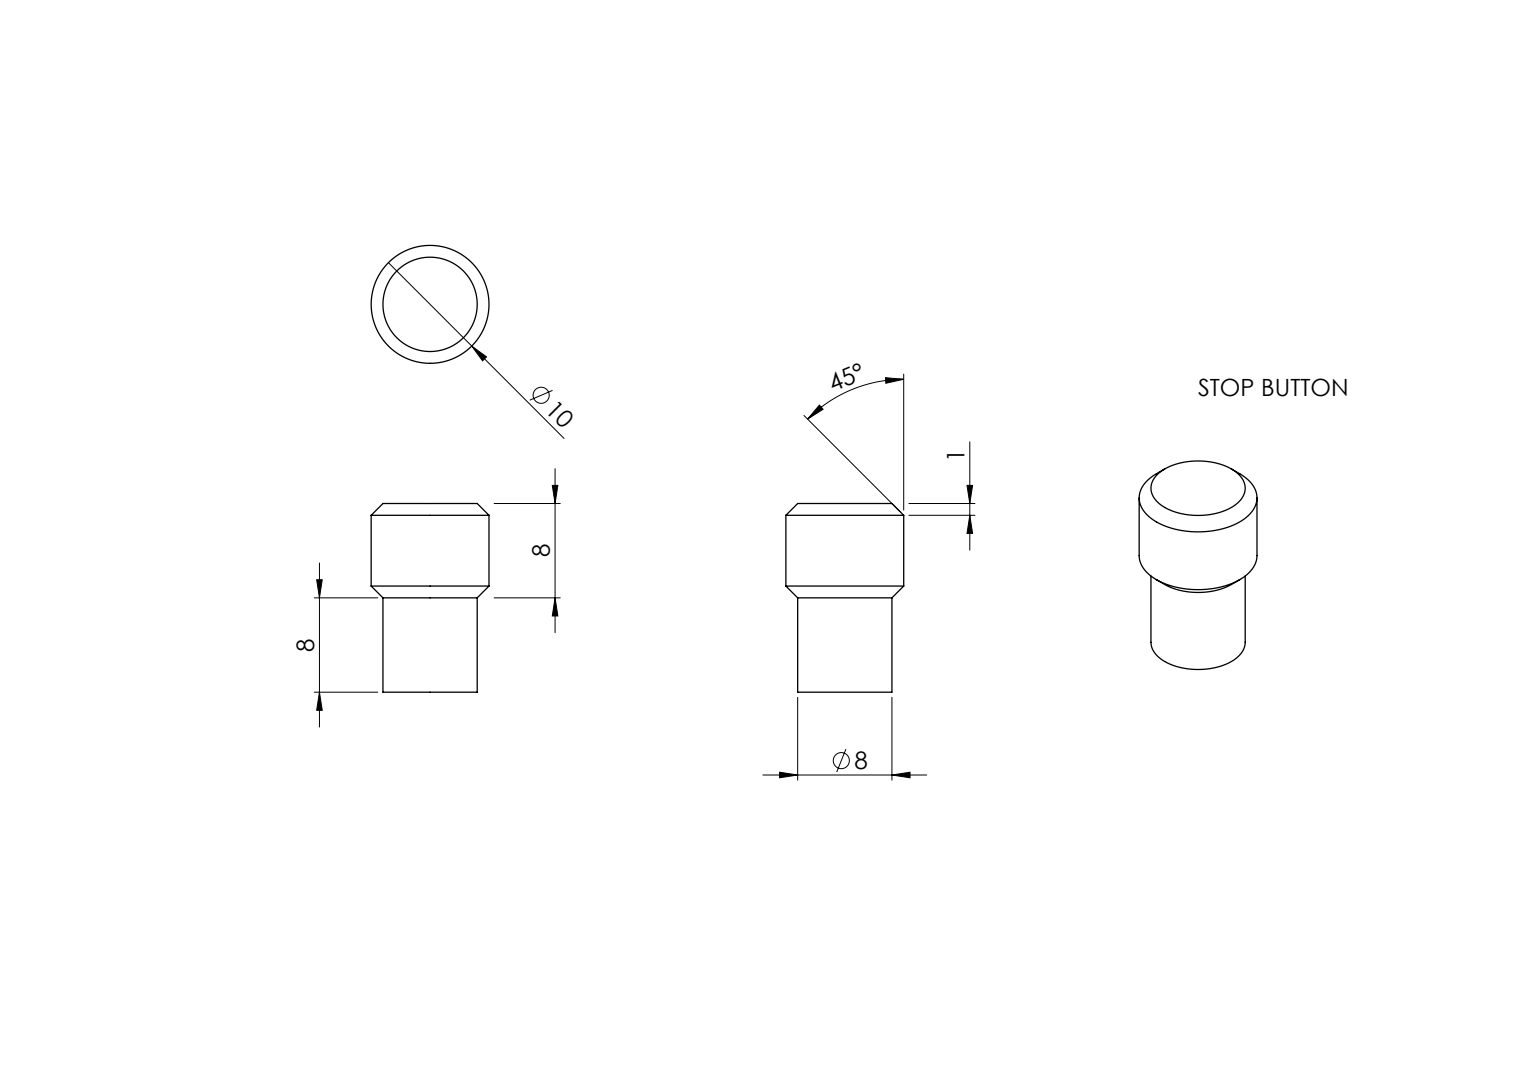
ISO-10303-21;
HEADER;
FILE_DESCRIPTION (('STEP AP214'),
    '1' );
FILE_NAME ('stop button.step',
    '2026-10-26T11:20:31',
    ( '' ),
    ( '' ),
    'SwSTEP 2.0',
    'SolidWorks 2026',
    '' );
FILE_SCHEMA (( 'AUTOMOTIVE_DESIGN' ));
ENDSEC;

DATA;
#2=ORIENTED_EDGE ( 'NONE', *, *, #1110, .F. ) ;
#22=VERTEX_POINT ( 'NONE', #4223 ) ;
#32=( LENGTH_UNIT ( ) NAMED_UNIT ( * ) SI_UNIT ( .MILLI., .METRE. ) );
#39=CIRCLE ( 'NONE', #1106, 4.000000000000000000 ) ;
#62=DIRECTION ( 'NONE',  ( 0.000000000000000000, 0.000000000000000000, 1.000000000000000000 ) ) ;
#65=DIRECTION ( 'NONE',  ( 0.000000000000000000, 1.000000000000000000, 0.000000000000000000 ) ) ;
#85=VERTEX_POINT ( 'NONE', #4577 ) ;
#123=DIRECTION ( 'NONE',  ( -0.000000000000000000, -1.000000000000000000, -0.000000000000000000 ) ) ;
#130=DIRECTION ( 'NONE',  ( 0.000000000000000000, 0.000000000000000000, 1.000000000000000000 ) ) ;
#135=PRODUCT_DEFINITION_FORMATION_WITH_SPECIFIED_SOURCE ( 'ANY', '', #1681, .NOT_KNOWN. ) ;
#149=ORIENTED_EDGE ( 'NONE', *, *, #4614, .F. ) ;
#153=UNCERTAINTY_MEASURE_WITH_UNIT (LENGTH_MEASURE( 1.000000000000000082E-05 ), #374, 'distance_accuracy_value', 'NONE');
#173=CIRCLE ( 'NONE', #776, 5.000000000000000888 ) ;
#201=FACE_OUTER_BOUND ( 'NONE', #427, .T. ) ;
#205=AXIS2_PLACEMENT_3D ( 'NONE', #2218, #4537, #1354 ) ;
#255=DIRECTION ( 'NONE',  ( 0.000000000000000000, 0.000000000000000000, 1.000000000000000000 ) ) ;
#282=ORIENTED_EDGE ( 'NONE', *, *, #4614, .T. ) ;
#288=PRODUCT_DEFINITION_CONTEXT ( 'detailed design', #920, 'design' ) ;
#308=CARTESIAN_POINT ( 'NONE',  ( 3.469446951953614189E-15, 34.00000000000000000, 8.999999999999992895 ) ) ;
#310=VERTEX_POINT ( 'NONE', #3063 ) ;
#320=PRODUCT_CONTEXT ( 'NONE', #3923, 'mechanical' ) ;
#323=DIRECTION ( 'NONE',  ( -0.000000000000000000, -1.000000000000000000, -0.000000000000000000 ) ) ;
#324=LINE ( 'NONE', #1796, #4294 ) ;
#352=CARTESIAN_POINT ( 'NONE',  ( 3.469446951953614189E-15, 41.00000000000000000, 8.999999999999992895 ) ) ;
#374=( LENGTH_UNIT ( ) NAMED_UNIT ( * ) SI_UNIT ( .MILLI., .METRE. ) );
#380=AXIS2_PLACEMENT_3D ( 'NONE', #2484, #3587, #1024 ) ;
#385=CARTESIAN_POINT ( 'NONE',  ( 3.469446951953614189E-15, 33.00000000000000000, 8.999999999999992895 ) ) ;
#397=( NAMED_UNIT ( * ) SI_UNIT ( $, .STERADIAN. ) SOLID_ANGLE_UNIT ( ) );
#403=DIRECTION ( 'NONE',  ( -0.000000000000000000, 1.000000000000000000, -0.000000000000000000 ) ) ;
#427=EDGE_LOOP ( 'NONE', ( #1515, #2000, #282, #1851 ) ) ;
#450=ORIENTED_EDGE ( 'NONE', *, *, #688, .F. ) ;
#473=SURFACE_STYLE_FILL_AREA ( #1539 ) ;
#578=( GEOMETRIC_REPRESENTATION_CONTEXT ( 3 ) GLOBAL_UNCERTAINTY_ASSIGNED_CONTEXT ( ( #4075 ) ) GLOBAL_UNIT_ASSIGNED_CONTEXT ( ( #32, #1473, #1933 ) ) REPRESENTATION_CONTEXT ( 'NONE', 'WORKASPACE' ) );
#580=DIRECTION ( 'NONE',  ( 0.000000000000000000, 1.000000000000000000, 0.000000000000000000 ) ) ;
#584=DIRECTION ( 'NONE',  ( -0.000000000000000000, -1.000000000000000000, -0.000000000000000000 ) ) ;
#592=MECHANICAL_DESIGN_GEOMETRIC_PRESENTATION_REPRESENTATION('',(#1718),#2469);
#617=DIRECTION ( 'NONE',  ( 0.000000000000000000, 0.000000000000000000, 1.000000000000000000 ) ) ;
#642=CARTESIAN_POINT ( 'NONE',  ( 3.469446951953614189E-15, 37.00000000000000711, 4.999999999999992006 ) ) ;
#688=EDGE_CURVE ( 'NONE', #2966, #22, #4307, .T. ) ;
#697=LINE ( 'NONE', #3186, #1821 ) ;
#759=ORIENTED_EDGE ( 'NONE', *, *, #4685, .T. ) ;
#776=AXIS2_PLACEMENT_3D ( 'NONE', #3918, #3873, #255 ) ;
#804=EDGE_CURVE ( 'NONE', #85, #3729, #1345, .T. ) ;
#865=DIRECTION ( 'NONE',  ( -0.000000000000000000, 1.000000000000000000, -0.000000000000000000 ) ) ;
#912=CARTESIAN_POINT ( 'NONE',  ( 3.469446951953614189E-15, 25.00000000000000000, 8.999999999999992895 ) ) ;
#916=EDGE_CURVE ( 'NONE', #22, #310, #1522, .T. ) ;
#920=APPLICATION_CONTEXT ( 'automotive_design' ) ;
#946=CYLINDRICAL_SURFACE ( 'NONE', #2530, 5.000000000000000888 ) ;
#957=ADVANCED_FACE ( 'NONE', ( #3302 ), #1952, .T. ) ;
#1002=DIRECTION ( 'NONE',  ( -0.000000000000000000, -1.000000000000000000, -0.000000000000000000 ) ) ;
#1021=ORIENTED_EDGE ( 'NONE', *, *, #4190, .F. ) ;
#1024=DIRECTION ( 'NONE',  ( 0.000000000000000000, -0.000000000000000000, 1.000000000000000000 ) ) ;
#1040=EDGE_CURVE ( 'NONE', #2780, #85, #1094, .T. ) ;
#1084=AXIS2_PLACEMENT_3D ( 'NONE', #2427, #2821, #2086 ) ;
#1094=LINE ( 'NONE', #4313, #1117 ) ;
#1106=AXIS2_PLACEMENT_3D ( 'NONE', #3743, #1553, #62 ) ;
#1110=EDGE_CURVE ( 'NONE', #3335, #4618, #1587, .T. ) ;
#1117=VECTOR ( 'NONE', #2486, 1000.000000000000000 ) ;
#1119=ORIENTED_EDGE ( 'NONE', *, *, #3787, .F. ) ;
#1164=( NAMED_UNIT ( * ) PLANE_ANGLE_UNIT ( ) SI_UNIT ( $, .RADIAN. ) );
#1172=CARTESIAN_POINT ( 'NONE',  ( 3.959305671612554781E-15, 41.00000000000000000, 12.99999999999999289 ) ) ;
#1173=ORIENTED_EDGE ( 'NONE', *, *, #1731, .F. ) ;
#1176=DIRECTION ( 'NONE',  ( 0.000000000000000000, 0.000000000000000000, 1.000000000000000000 ) ) ;
#1191=CARTESIAN_POINT ( 'NONE',  ( 3.469446951953614189E-15, 25.00000000000000000, 4.999999999999992006 ) ) ;
#1222=DIRECTION ( 'NONE',  ( 0.000000000000000000, 0.000000000000000000, 1.000000000000000000 ) ) ;
#1230=CARTESIAN_POINT ( 'NONE',  ( 3.469446951953614189E-15, 33.00000000000000000, 8.999999999999992895 ) ) ;
#1239=VERTEX_POINT ( 'NONE', #1191 ) ;
#1242=ORIENTED_EDGE ( 'NONE', *, *, #1620, .T. ) ;
#1321=CARTESIAN_POINT ( 'NONE',  ( 3.959305671612554781E-15, 25.00000000000000000, 12.99999999999999289 ) ) ;
#1337=AXIS2_PLACEMENT_3D ( 'NONE', #3194, #2076, #2167 ) ;
#1338=ORIENTED_EDGE ( 'NONE', *, *, #4058, .T. ) ;
#1345=CIRCLE ( 'NONE', #1947, 5.000000000000000888 ) ;
#1354=DIRECTION ( 'NONE',  ( 0.000000000000000000, 0.000000000000000000, 1.000000000000000000 ) ) ;
#1384=VECTOR ( 'NONE', #323, 1000.000000000000000 ) ;
#1388=ADVANCED_FACE ( 'NONE', ( #3563 ), #3167, .T. ) ;
#1399=EDGE_CURVE ( 'NONE', #310, #3729, #697, .T. ) ;
#1415=ADVANCED_FACE ( 'NONE', ( #1800 ), #2438, .F. ) ;
#1421=EDGE_LOOP ( 'NONE', ( #1338, #2203, #4426, #149 ) ) ;
#1426=ORIENTED_EDGE ( 'NONE', *, *, #1764, .F. ) ;
#1473=( NAMED_UNIT ( * ) PLANE_ANGLE_UNIT ( ) SI_UNIT ( $, .RADIAN. ) );
#1486=EDGE_LOOP ( 'NONE', ( #4239, #3021, #2201, #1426 ) ) ;
#1515=ORIENTED_EDGE ( 'NONE', *, *, #3618, .F. ) ;
#1522=LINE ( 'NONE', #1172, #2936 ) ;
#1539=FILL_AREA_STYLE ('',( #3348 ) ) ;
#1553=DIRECTION ( 'NONE',  ( 0.000000000000000000, 1.000000000000000000, 0.000000000000000000 ) ) ;
#1587=LINE ( 'NONE', #3018, #4415 ) ;
#1620=EDGE_CURVE ( 'NONE', #2966, #2780, #3749, .T. ) ;
#1621=LINE ( 'NONE', #3073, #3384 ) ;
#1636=ORIENTED_EDGE ( 'NONE', *, *, #1764, .T. ) ;
#1681=PRODUCT ( 'stop button', 'stop button', '', ( #320 ) ) ;
#1694=CARTESIAN_POINT ( 'NONE',  ( 3.469446951953614189E-15, 41.00000000000000000, 8.999999999999992895 ) ) ;
#1695=FACE_OUTER_BOUND ( 'NONE', #2068, .T. ) ;
#1701=AXIS2_PLACEMENT_3D ( 'NONE', #385, #2284, #1176 ) ;
#1709=EDGE_LOOP ( 'NONE', ( #1911, #4314 ) ) ;
#1712=DIRECTION ( 'NONE',  ( 0.000000000000000000, 0.000000000000000000, 1.000000000000000000 ) ) ;
#1715=FACE_OUTER_BOUND ( 'NONE', #1486, .T. ) ;
#1718=STYLED_ITEM ( 'NONE', ( #2222 ), #3296 ) ;
#1731=EDGE_CURVE ( 'NONE', #310, #2780, #173, .T. ) ;
#1764=EDGE_CURVE ( 'NONE', #2296, #1239, #2774, .T. ) ;
#1776=AXIS2_PLACEMENT_3D ( 'NONE', #1841, #4643, #3947 ) ;
#1780=CARTESIAN_POINT ( 'NONE',  ( 0.000000000000000000, 0.000000000000000000, 0.000000000000000000 ) ) ;
#1790=EDGE_CURVE ( 'NONE', #2780, #310, #2592, .T. ) ;
#1796=CARTESIAN_POINT ( 'NONE',  ( 4.081770351527290718E-15, 34.00000000000000000, 3.999999999999991562 ) ) ;
#1800=FACE_OUTER_BOUND ( 'NONE', #1709, .T. ) ;
#1811=FACE_OUTER_BOUND ( 'NONE', #2919, .T. ) ;
#1821=VECTOR ( 'NONE', #1002, 1000.000000000000000 ) ;
#1826=ORIENTED_EDGE ( 'NONE', *, *, #1399, .F. ) ;
#1841=CARTESIAN_POINT ( 'NONE',  ( 3.469446951953614189E-15, 37.00000000000000711, 8.999999999999992895 ) ) ;
#1851=ORIENTED_EDGE ( 'NONE', *, *, #804, .F. ) ;
#1887=AXIS2_PLACEMENT_3D ( 'NONE', #3733, #1931, #4103 ) ;
#1900=( NAMED_UNIT ( * ) PLANE_ANGLE_UNIT ( ) SI_UNIT ( $, .RADIAN. ) );
#1911=ORIENTED_EDGE ( 'NONE', *, *, #4685, .F. ) ;
#1913=DIRECTION ( 'NONE',  ( 0.000000000000000000, 0.000000000000000000, 1.000000000000000000 ) ) ;
#1917=CLOSED_SHELL ( 'NONE', ( #4383, #957, #3287, #2257, #3724, #1415, #4263, #1388, #2101, #2629 ) ) ;
#1925=SURFACE_STYLE_USAGE ( .BOTH. , #2992 ) ;
#1931=DIRECTION ( 'NONE',  ( 0.000000000000000000, -1.000000000000000000, 0.000000000000000000 ) ) ;
#1933=( NAMED_UNIT ( * ) SI_UNIT ( $, .STERADIAN. ) SOLID_ANGLE_UNIT ( ) );
#1947=AXIS2_PLACEMENT_3D ( 'NONE', #2746, #3509, #617 ) ;
#1948=DIRECTION ( 'NONE',  ( 0.000000000000000000, -0.7071067811865500152, -0.7071067811865451302 ) ) ;
#1952=CONICAL_SURFACE ( 'NONE', #4535, 5.000000000000000888, 0.7853981633974517207 ) ;
#1973=CARTESIAN_POINT ( 'NONE',  ( 3.469446951953614189E-15, 41.00000000000000000, 4.999999999999992006 ) ) ;
#2000=ORIENTED_EDGE ( 'NONE', *, *, #3787, .T. ) ;
#2021=EDGE_CURVE ( 'NONE', #3729, #85, #2144, .T. ) ;
#2023=CARTESIAN_POINT ( 'NONE',  ( 3.469446951953614189E-15, 39.99999999999999289, 3.999999999999991562 ) ) ;
#2034=DIRECTION ( 'NONE',  ( 0.000000000000000000, 0.000000000000000000, -1.000000000000000000 ) ) ;
#2035=CARTESIAN_POINT ( 'NONE',  ( 3.469446951953614189E-15, 41.00000000000000000, 8.999999999999992895 ) ) ;
#2046=ORIENTED_EDGE ( 'NONE', *, *, #916, .F. ) ;
#2053=DIRECTION ( 'NONE',  ( 0.000000000000000000, 0.000000000000000000, -1.000000000000000000 ) ) ;
#2068=EDGE_LOOP ( 'NONE', ( #1826, #2219, #2281, #4645 ) ) ;
#2072=DIRECTION ( 'NONE',  ( 0.000000000000000000, 1.000000000000000000, 0.000000000000000000 ) ) ;
#2076=DIRECTION ( 'NONE',  ( 0.000000000000000000, -1.000000000000000000, 0.000000000000000000 ) ) ;
#2086=DIRECTION ( 'NONE',  ( 0.000000000000000000, 0.000000000000000000, 1.000000000000000000 ) ) ;
#2101=ADVANCED_FACE ( 'NONE', ( #201 ), #3972, .T. ) ;
#2107=DIRECTION ( 'NONE',  ( 8.659560562354962440E-17, 0.7071067811865451302, -0.7071067811865500152 ) ) ;
#2132=CARTESIAN_POINT ( 'NONE',  ( 4.081770351527290718E-15, 34.00000000000000000, 13.99999999999999289 ) ) ;
#2144=CIRCLE ( 'NONE', #3510, 5.000000000000000888 ) ;
#2167=DIRECTION ( 'NONE',  ( 0.000000000000000000, 0.000000000000000000, -1.000000000000000000 ) ) ;
#2201=ORIENTED_EDGE ( 'NONE', *, *, #4620, .T. ) ;
#2202=ORIENTED_EDGE ( 'NONE', *, *, #1790, .T. ) ;
#2203=ORIENTED_EDGE ( 'NONE', *, *, #3618, .T. ) ;
#2218=CARTESIAN_POINT ( 'NONE',  ( 3.469446951953614189E-15, 41.00000000000000000, 8.999999999999992895 ) ) ;
#2219=ORIENTED_EDGE ( 'NONE', *, *, #1731, .T. ) ;
#2222=PRESENTATION_STYLE_ASSIGNMENT (( #1925 ) ) ;
#2257=ADVANCED_FACE ( 'NONE', ( #1715 ), #2739, .T. ) ;
#2271=EDGE_LOOP ( 'NONE', ( #2202, #3045, #4249, #2708 ) ) ;
#2277=FACE_OUTER_BOUND ( 'NONE', #3350, .T. ) ;
#2281=ORIENTED_EDGE ( 'NONE', *, *, #1040, .T. ) ;
#2284=DIRECTION ( 'NONE',  ( 0.000000000000000000, 1.000000000000000000, 0.000000000000000000 ) ) ;
#2296=VERTEX_POINT ( 'NONE', #4225 ) ;
#2309=DIRECTION ( 'NONE',  ( 0.000000000000000000, 0.000000000000000000, 1.000000000000000000 ) ) ;
#2374=CIRCLE ( 'NONE', #3453, 4.000000000000000000 ) ;
#2404=CONICAL_SURFACE ( 'NONE', #1887, 4.000000000000000000, 0.7853981633974447263 ) ;
#2424=AXIS2_PLACEMENT_3D ( 'NONE', #352, #3879, #4623 ) ;
#2427=CARTESIAN_POINT ( 'NONE',  ( 3.469446951953614189E-15, 39.99999999999999289, 8.999999999999992895 ) ) ;
#2434=EDGE_LOOP ( 'NONE', ( #3140, #4533 ) ) ;
#2438=PLANE ( 'NONE',  #380 ) ;
#2456=CIRCLE ( 'NONE', #4607, 4.000000000000000000 ) ;
#2469=( GEOMETRIC_REPRESENTATION_CONTEXT ( 3 ) GLOBAL_UNCERTAINTY_ASSIGNED_CONTEXT ( ( #153 ) ) GLOBAL_UNIT_ASSIGNED_CONTEXT ( ( #374, #1164, #397 ) ) REPRESENTATION_CONTEXT ( 'NONE', 'WORKASPACE' ) );
#2477=CYLINDRICAL_SURFACE ( 'NONE', #1776, 4.000000000000000000 ) ;
#2484=CARTESIAN_POINT ( 'NONE',  ( 3.469446951953614189E-15, 25.00000000000000000, 8.999999999999992895 ) ) ;
#2486=DIRECTION ( 'NONE',  ( -0.000000000000000000, -1.000000000000000000, -0.000000000000000000 ) ) ;
#2514=AXIS2_PLACEMENT_3D ( 'NONE', #4109, #865, #1913 ) ;
#2530=AXIS2_PLACEMENT_3D ( 'NONE', #2035, #2668, #2053 ) ;
#2539=CARTESIAN_POINT ( 'NONE',  ( 3.959305671612554781E-15, 33.00000000000000000, 12.99999999999999289 ) ) ;
#2543=( GEOMETRIC_REPRESENTATION_CONTEXT ( 3 ) GLOBAL_UNCERTAINTY_ASSIGNED_CONTEXT ( ( #3760 ) ) GLOBAL_UNIT_ASSIGNED_CONTEXT ( ( #4398, #1900, #2555 ) ) REPRESENTATION_CONTEXT ( 'NONE', 'WORKASPACE' ) );
#2555=( NAMED_UNIT ( * ) SI_UNIT ( $, .STERADIAN. ) SOLID_ANGLE_UNIT ( ) );
#2592=CIRCLE ( 'NONE', #1084, 5.000000000000000888 ) ;
#2596=AXIS2_PLACEMENT_3D ( 'NONE', #3192, #584, #2034 ) ;
#2629=ADVANCED_FACE ( 'NONE', ( #2277 ), #2404, .T. ) ;
#2668=DIRECTION ( 'NONE',  ( -0.000000000000000000, -1.000000000000000000, -0.000000000000000000 ) ) ;
#2708=ORIENTED_EDGE ( 'NONE', *, *, #1040, .F. ) ;
#2739=CYLINDRICAL_SURFACE ( 'NONE', #2596, 4.000000000000000000 ) ;
#2746=CARTESIAN_POINT ( 'NONE',  ( 3.469446951953614189E-15, 34.00000000000000000, 8.999999999999992895 ) ) ;
#2774=LINE ( 'NONE', #642, #1384 ) ;
#2780=VERTEX_POINT ( 'NONE', #2023 ) ;
#2790=DIRECTION ( 'NONE',  ( -0.000000000000000000, -1.000000000000000000, -0.000000000000000000 ) ) ;
#2821=DIRECTION ( 'NONE',  ( 0.000000000000000000, -1.000000000000000000, 0.000000000000000000 ) ) ;
#2823=PRODUCT_DEFINITION_SHAPE ( 'NONE', 'NONE',  #2956 ) ;
#2846=FACE_OUTER_BOUND ( 'NONE', #2902, .T. ) ;
#2899=VECTOR ( 'NONE', #1948, 1000.000000000000114 ) ;
#2902=EDGE_LOOP ( 'NONE', ( #2, #1119, #1636, #759 ) ) ;
#2919=EDGE_LOOP ( 'NONE', ( #1021, #3951, #4519, #4424 ) ) ;
#2928=AXIS2_PLACEMENT_3D ( 'NONE', #1780, #1712, #3957 ) ;
#2936=VECTOR ( 'NONE', #2977, 1000.000000000000114 ) ;
#2956=PRODUCT_DEFINITION ( 'UNKNOWN', '', #135, #288 ) ;
#2960=CARTESIAN_POINT ( 'NONE',  ( 3.469446951953614189E-15, 41.00000000000000000, 4.999999999999992006 ) ) ;
#2966=VERTEX_POINT ( 'NONE', #2960 ) ;
#2977=DIRECTION ( 'NONE',  ( 8.659560562354903276E-17, -0.7071067811865500152, 0.7071067811865451302 ) ) ;
#2992=SURFACE_SIDE_STYLE ('',( #473 ) ) ;
#3018=CARTESIAN_POINT ( 'NONE',  ( 3.959305671612554781E-15, 37.00000000000000711, 12.99999999999999289 ) ) ;
#3021=ORIENTED_EDGE ( 'NONE', *, *, #1110, .T. ) ;
#3045=ORIENTED_EDGE ( 'NONE', *, *, #1399, .T. ) ;
#3063=CARTESIAN_POINT ( 'NONE',  ( 4.081770351527290718E-15, 39.99999999999999289, 13.99999999999999289 ) ) ;
#3073=CARTESIAN_POINT ( 'NONE',  ( 3.469446951953614189E-15, 34.00000000000000000, 13.99999999999999289 ) ) ;
#3140=ORIENTED_EDGE ( 'NONE', *, *, #688, .T. ) ;
#3143=CARTESIAN_POINT ( 'NONE',  ( 3.469446951953614189E-15, 25.00000000000000000, 8.999999999999992895 ) ) ;
#3161=COLOUR_RGB ( '',0.8941176470588234615, 0.8941176470588234615, 0.8941176470588234615 ) ;
#3167=PLANE ( 'NONE',  #2424 ) ;
#3184=AXIS2_PLACEMENT_3D ( 'NONE', #1694, #2790, #3884 ) ;
#3186=CARTESIAN_POINT ( 'NONE',  ( 4.081770351527290718E-15, 41.00000000000000000, 13.99999999999999289 ) ) ;
#3192=CARTESIAN_POINT ( 'NONE',  ( 3.469446951953614189E-15, 37.00000000000000711, 8.999999999999992895 ) ) ;
#3194=CARTESIAN_POINT ( 'NONE',  ( 3.469446951953614189E-15, 41.00000000000000000, 8.999999999999992895 ) ) ;
#3210=DIRECTION ( 'NONE',  ( 0.000000000000000000, 0.000000000000000000, 1.000000000000000000 ) ) ;
#3257=DIRECTION ( 'NONE',  ( -0.000000000000000000, 1.000000000000000000, -0.000000000000000000 ) ) ;
#3287=ADVANCED_FACE ( 'NONE', ( #4704 ), #3501, .T. ) ;
#3296=ADVANCED_BREP_SHAPE_REPRESENTATION ( '', ( #4442, #2928 ), #2543 ) ;
#3301=CIRCLE ( 'NONE', #3912, 4.000000000000000000 ) ;
#3302=FACE_OUTER_BOUND ( 'NONE', #1421, .T. ) ;
#3335=VERTEX_POINT ( 'NONE', #2539 ) ;
#3348=FILL_AREA_STYLE_COLOUR ( '', #3161 ) ;
#3350=EDGE_LOOP ( 'NONE', ( #2046, #450, #1242, #1173 ) ) ;
#3378=CARTESIAN_POINT ( 'NONE',  ( 3.469446951953614189E-15, 34.00000000000000000, 8.999999999999992895 ) ) ;
#3379=CONICAL_SURFACE ( 'NONE', #1337, 4.000000000000000000, 0.7853981633974447263 ) ;
#3384=VECTOR ( 'NONE', #4528, 1000.000000000000114 ) ;
#3453=AXIS2_PLACEMENT_3D ( 'NONE', #1230, #65, #2309 ) ;
#3462=STYLED_ITEM('',(#4729),#4442);
#3501=CYLINDRICAL_SURFACE ( 'NONE', #3184, 5.000000000000000888 ) ;
#3509=DIRECTION ( 'NONE',  ( -0.000000000000000000, 1.000000000000000000, -0.000000000000000000 ) ) ;
#3510=AXIS2_PLACEMENT_3D ( 'NONE', #3378, #403, #130 ) ;
#3563=FACE_OUTER_BOUND ( 'NONE', #2434, .T. ) ;
#3587=DIRECTION ( 'NONE',  ( 0.000000000000000000, 1.000000000000000000, 0.000000000000000000 ) ) ;
#3603=CIRCLE ( 'NONE', #1701, 4.000000000000000000 ) ;
#3618=EDGE_CURVE ( 'NONE', #2296, #85, #324, .T. ) ;
#3656=SHAPE_REPRESENTATION_RELATIONSHIP ( 'NONE' , 'NONE' ,  #3681, #3296 ) ;
#3681=SHAPE_REPRESENTATION ( 'stop button', ( #2928 ), #2543 ) ;
#3724=ADVANCED_FACE ( 'NONE', ( #2846 ), #2477, .T. ) ;
#3729=VERTEX_POINT ( 'NONE', #2132 ) ;
#3733=CARTESIAN_POINT ( 'NONE',  ( 3.469446951953614189E-15, 41.00000000000000000, 8.999999999999992895 ) ) ;
#3743=CARTESIAN_POINT ( 'NONE',  ( 3.469446951953614189E-15, 41.00000000000000000, 8.999999999999992895 ) ) ;
#3749=LINE ( 'NONE', #1973, #2899 ) ;
#3760=UNCERTAINTY_MEASURE_WITH_UNIT (LENGTH_MEASURE( 1.000000000000000082E-05 ), #4398, 'distance_accuracy_value', 'NONE');
#3787=EDGE_CURVE ( 'NONE', #2296, #3335, #2374, .T. ) ;
#3873=DIRECTION ( 'NONE',  ( 0.000000000000000000, -1.000000000000000000, 0.000000000000000000 ) ) ;
#3879=DIRECTION ( 'NONE',  ( 0.000000000000000000, 1.000000000000000000, 0.000000000000000000 ) ) ;
#3884=DIRECTION ( 'NONE',  ( 0.000000000000000000, 0.000000000000000000, -1.000000000000000000 ) ) ;
#3912=AXIS2_PLACEMENT_3D ( 'NONE', #912, #580, #1222 ) ;
#3918=CARTESIAN_POINT ( 'NONE',  ( 3.469446951953614189E-15, 39.99999999999999289, 8.999999999999992895 ) ) ;
#3923=APPLICATION_CONTEXT ( 'automotive_design' ) ;
#3931=DIRECTION ( 'NONE',  ( 0.000000000000000000, 0.000000000000000000, 1.000000000000000000 ) ) ;
#3947=DIRECTION ( 'NONE',  ( 0.000000000000000000, 0.000000000000000000, -1.000000000000000000 ) ) ;
#3951=ORIENTED_EDGE ( 'NONE', *, *, #916, .T. ) ;
#3957=DIRECTION ( 'NONE',  ( 1.000000000000000000, 0.000000000000000000, 0.000000000000000000 ) ) ;
#3972=CONICAL_SURFACE ( 'NONE', #2514, 5.000000000000000888, 0.7853981633974517207 ) ;
#4058=EDGE_CURVE ( 'NONE', #3335, #2296, #3603, .T. ) ;
#4075=UNCERTAINTY_MEASURE_WITH_UNIT (LENGTH_MEASURE( 1.000000000000000082E-05 ), #32, 'distance_accuracy_value', 'NONE');
#4103=DIRECTION ( 'NONE',  ( 0.000000000000000000, 0.000000000000000000, -1.000000000000000000 ) ) ;
#4109=CARTESIAN_POINT ( 'NONE',  ( 3.469446951953614189E-15, 34.00000000000000000, 8.999999999999992895 ) ) ;
#4190=EDGE_CURVE ( 'NONE', #22, #2966, #39, .T. ) ;
#4223=CARTESIAN_POINT ( 'NONE',  ( 4.020538011569923144E-15, 41.00000000000000000, 12.99999999999999289 ) ) ;
#4225=CARTESIAN_POINT ( 'NONE',  ( 3.469446951953614189E-15, 33.00000000000000000, 4.999999999999992006 ) ) ;
#4239=ORIENTED_EDGE ( 'NONE', *, *, #4058, .F. ) ;
#4249=ORIENTED_EDGE ( 'NONE', *, *, #2021, .T. ) ;
#4263=ADVANCED_FACE ( 'NONE', ( #1695 ), #946, .T. ) ;
#4294=VECTOR ( 'NONE', #2107, 1000.000000000000114 ) ;
#4298=MECHANICAL_DESIGN_GEOMETRIC_PRESENTATION_REPRESENTATION('',(#3462),#578);
#4300=SHAPE_DEFINITION_REPRESENTATION ( #2823, #3681 ) ;
#4307=CIRCLE ( 'NONE', #205, 4.000000000000000000 ) ;
#4313=CARTESIAN_POINT ( 'NONE',  ( 3.469446951953614189E-15, 41.00000000000000000, 3.999999999999991562 ) ) ;
#4314=ORIENTED_EDGE ( 'NONE', *, *, #4620, .F. ) ;
#4383=ADVANCED_FACE ( 'NONE', ( #1811 ), #3379, .T. ) ;
#4398=( LENGTH_UNIT ( ) NAMED_UNIT ( * ) SI_UNIT ( .MILLI., .METRE. ) );
#4415=VECTOR ( 'NONE', #123, 1000.000000000000000 ) ;
#4424=ORIENTED_EDGE ( 'NONE', *, *, #1620, .F. ) ;
#4426=ORIENTED_EDGE ( 'NONE', *, *, #2021, .F. ) ;
#4442=MANIFOLD_SOLID_BREP ( 'Chamfer1', #1917 ) ;
#4519=ORIENTED_EDGE ( 'NONE', *, *, #1790, .F. ) ;
#4528=DIRECTION ( 'NONE',  ( 0.000000000000000000, 0.7071067811865451302, 0.7071067811865500152 ) ) ;
#4533=ORIENTED_EDGE ( 'NONE', *, *, #4190, .T. ) ;
#4535=AXIS2_PLACEMENT_3D ( 'NONE', #308, #3257, #3210 ) ;
#4537=DIRECTION ( 'NONE',  ( 0.000000000000000000, 1.000000000000000000, 0.000000000000000000 ) ) ;
#4577=CARTESIAN_POINT ( 'NONE',  ( 3.469446951953614189E-15, 34.00000000000000000, 3.999999999999991562 ) ) ;
#4607=AXIS2_PLACEMENT_3D ( 'NONE', #3143, #2072, #3931 ) ;
#4614=EDGE_CURVE ( 'NONE', #3335, #3729, #1621, .T. ) ;
#4618=VERTEX_POINT ( 'NONE', #1321 ) ;
#4620=EDGE_CURVE ( 'NONE', #4618, #1239, #3301, .T. ) ;
#4623=DIRECTION ( 'NONE',  ( 0.000000000000000000, -0.000000000000000000, 1.000000000000000000 ) ) ;
#4643=DIRECTION ( 'NONE',  ( -0.000000000000000000, -1.000000000000000000, -0.000000000000000000 ) ) ;
#4645=ORIENTED_EDGE ( 'NONE', *, *, #804, .T. ) ;
#4685=EDGE_CURVE ( 'NONE', #1239, #4618, #2456, .T. ) ;
#4704=FACE_OUTER_BOUND ( 'NONE', #2271, .T. ) ;
#4723=COLOUR_RGB('Light Blue',0.38,0.62,0.78);
#4724=FILL_AREA_STYLE_COLOUR('',#4723);
#4725=FILL_AREA_STYLE('',(#4724));
#4726=SURFACE_STYLE_FILL_AREA(#4725);
#4727=SURFACE_SIDE_STYLE('',(#4726));
#4728=SURFACE_STYLE_USAGE(.BOTH.,#4727);
#4729=PRESENTATION_STYLE_ASSIGNMENT((#4728));
ENDSEC;
END-ISO-10303-21;
